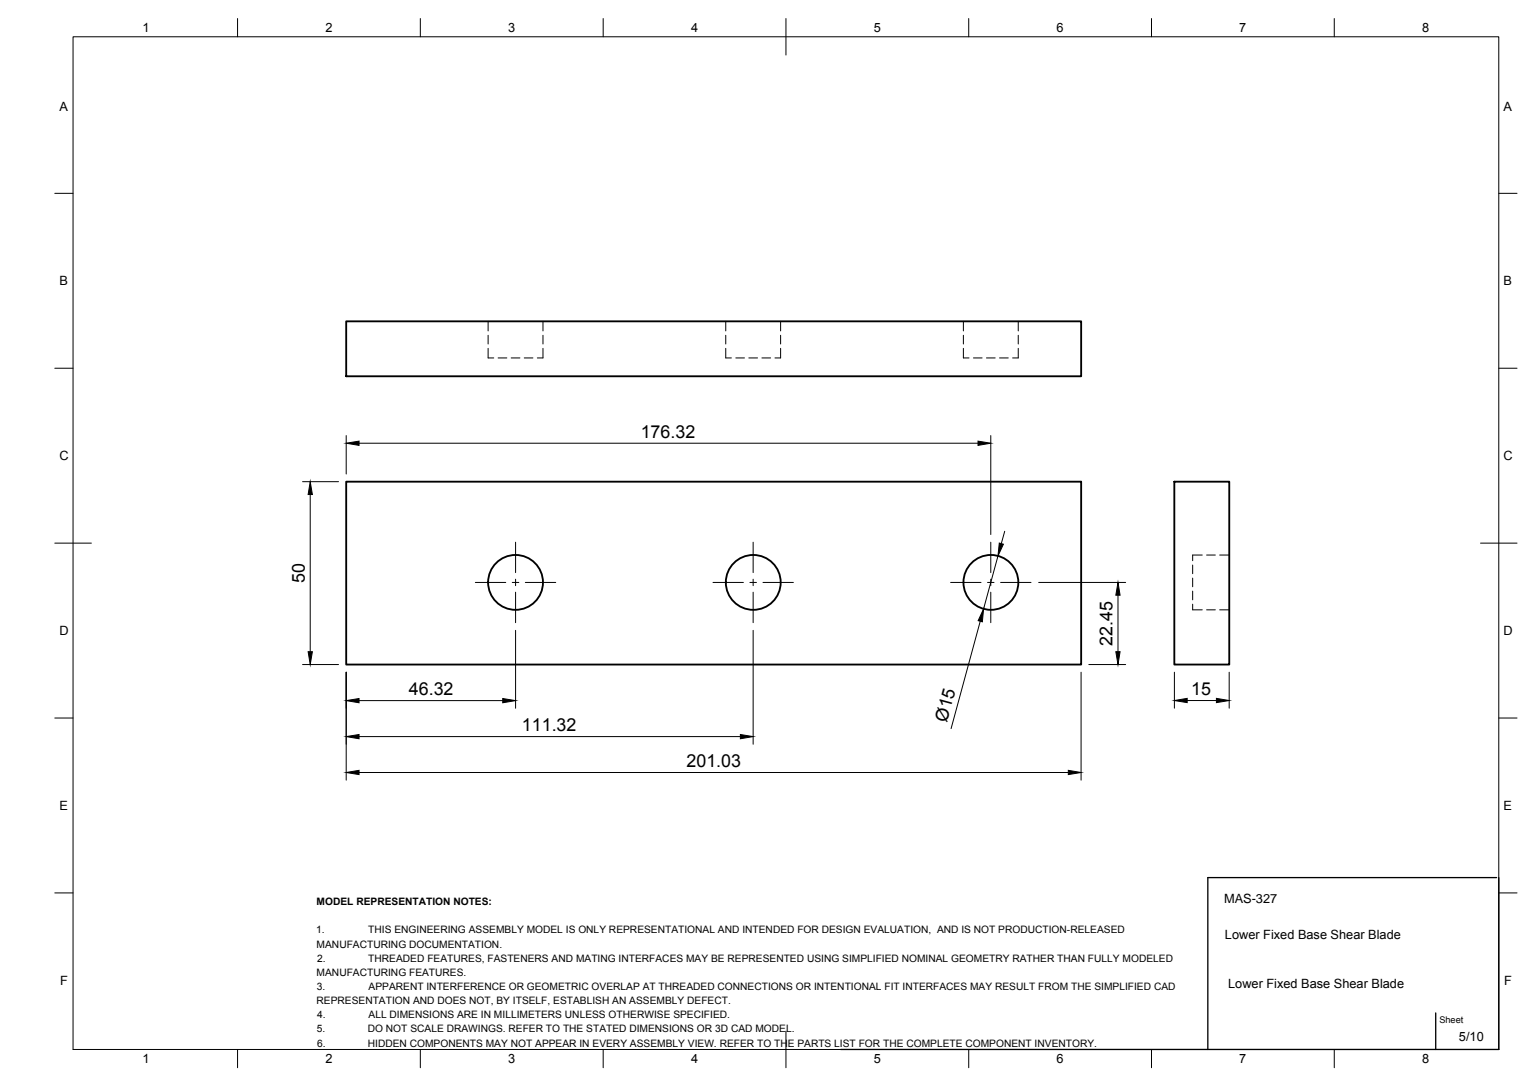
ISO-10303-21;
HEADER;
FILE_DESCRIPTION (('STEP AP214'),
    '1' );
FILE_NAME ('Lower Fixed Base Shear Blade.step',
    '2026-10-06T22:16:42',
    ( '' ),
    ( '' ),
    'SwSTEP 2.0',
    'SolidWorks 2025',
    '' );
FILE_SCHEMA (( 'AUTOMOTIVE_DESIGN' ));
ENDSEC;

DATA;
#67=AXIS2_PLACEMENT_3D ( 'NONE', #12131, #8413, #1572 ) ;
#82=DIRECTION ( 'NONE',  ( 0.000000000000000000, 0.000000000000000000, -1.000000000000000000 ) ) ;
#121=EDGE_CURVE ( 'NONE', #811, #5132, #2980, .T. ) ;
#220=CARTESIAN_POINT ( 'NONE',  ( 83.67254549292280785, -61.68114226949890622, 10.00000000000001599 ) ) ;
#222=ORIENTED_EDGE ( 'NONE', *, *, #8399, .T. ) ;
#275=CARTESIAN_POINT ( 'NONE',  ( 173.3794444120442506, -34.13255853780189142, 5.000000000000018652 ) ) ;
#342=EDGE_CURVE ( 'NONE', #19257, #8316, #5649, .T. ) ;
#343=( GEOMETRIC_REPRESENTATION_CONTEXT ( 3 ) GLOBAL_UNCERTAINTY_ASSIGNED_CONTEXT ( ( #15680 ) ) GLOBAL_UNIT_ASSIGNED_CONTEXT ( ( #12211, #2186, #7269 ) ) REPRESENTATION_CONTEXT ( 'NONE', 'WORKASPACE' ) );
#363=CARTESIAN_POINT ( 'NONE',  ( 18.67254549292281496, -61.68114226949890622, 10.00000000000001599 ) ) ;
#364=EDGE_CURVE ( 'NONE', #13608, #15461, #11277, .T. ) ;
#394=LINE ( 'NONE', #7017, #18876 ) ;
#660=EDGE_CURVE ( 'NONE', #15106, #2386, #14957, .T. ) ;
#672=LINE ( 'NONE', #7408, #19081 ) ;
#751=DIRECTION ( 'NONE',  ( 1.000000000000000000, 0.000000000000000000, 0.000000000000000000 ) ) ;
#771=AXIS2_PLACEMENT_3D ( 'NONE', #11380, #1580, #9853 ) ;
#811=VERTEX_POINT ( 'NONE', #13743 ) ;
#889=DIRECTION ( 'NONE',  ( 1.000000000000000000, -0.000000000000000000, -0.000000000000000000 ) ) ;
#892=EDGE_LOOP ( 'NONE', ( #21201, #9511, #8668, #6236 ) ) ;
#909=CARTESIAN_POINT ( 'NONE',  ( -27.64582385433944367, -84.13255853780189852, 5.000000000000018652 ) ) ;
#912=EDGE_LOOP ( 'NONE', ( #15164, #18877, #13960, #16804 ) ) ;
#919=CARTESIAN_POINT ( 'NONE',  ( 5.130598475945862827E-15, 0.000000000000000000, 20.00000000000001776 ) ) ;
#928=AXIS2_PLACEMENT_3D ( 'NONE', #10600, #15343, #18757 ) ;
#1190=PLANE ( 'NONE',  #6786 ) ;
#1247=FACE_OUTER_BOUND ( 'NONE', #20004, .T. ) ;
#1249=VERTEX_POINT ( 'NONE', #14943 ) ;
#1316=CARTESIAN_POINT ( 'NONE',  ( 18.67254549292281496, -61.68114226949890622, -16.21320343559643717 ) ) ;
#1428=CYLINDRICAL_SURFACE ( 'NONE', #9034, 7.500000000000000000 ) ;
#1449=ORIENTED_EDGE ( 'NONE', *, *, #19445, .T. ) ;
#1456=CARTESIAN_POINT ( 'NONE',  ( 83.67254549292280785, -61.68114226949890622, -16.21320343559643717 ) ) ;
#1481=CIRCLE ( 'NONE', #2895, 7.500000000000000000 ) ;
#1565=CIRCLE ( 'NONE', #17047, 7.500000000000007105 ) ;
#1572=DIRECTION ( 'NONE',  ( -1.000000000000000000, 0.000000000000000000, 0.000000000000000000 ) ) ;
#1580=DIRECTION ( 'NONE',  ( -0.000000000000000000, 0.000000000000000000, -1.000000000000000000 ) ) ;
#1638=DIRECTION ( 'NONE',  ( -0.000000000000000000, -0.000000000000000000, 1.000000000000000000 ) ) ;
#1724=FACE_OUTER_BOUND ( 'NONE', #3351, .T. ) ;
#1788=CARTESIAN_POINT ( 'NONE',  ( -27.64582385433943656, -34.13255853780189142, 5.000000000000018652 ) ) ;
#1876=DIRECTION ( 'NONE',  ( -0.000000000000000000, -0.000000000000000000, -1.000000000000000000 ) ) ;
#1912=CARTESIAN_POINT ( 'NONE',  ( 173.3794444120442506, -34.13255853780189142, 5.000000000000018652 ) ) ;
#2073=ORIENTED_EDGE ( 'NONE', *, *, #13532, .T. ) ;
#2131=CLOSED_SHELL ( 'NONE', ( #14070, #2497, #19372, #16215, #5248, #3409, #5840, #17907, #3304, #2907, #15780, #10582, #17008, #14366, #6702 ) ) ;
#2151=FILL_AREA_STYLE_COLOUR ( '', #21717 ) ;
#2186=( NAMED_UNIT ( * ) PLANE_ANGLE_UNIT ( ) SI_UNIT ( $, .RADIAN. ) );
#2350=STYLED_ITEM ( 'NONE', ( #2362 ), #14370 ) ;
#2362=PRESENTATION_STYLE_ASSIGNMENT (( #17561 ) ) ;
#2386=VERTEX_POINT ( 'NONE', #5094 ) ;
#2403=CARTESIAN_POINT ( 'NONE',  ( 0.000000000000000000, 0.000000000000000000, 0.000000000000000000 ) ) ;
#2410=DIRECTION ( 'NONE',  ( 1.387778780781445676E-16, 1.000000000000000000, -0.000000000000000000 ) ) ;
#2433=CARTESIAN_POINT ( 'NONE',  ( 173.3794444120442506, -34.13255853780189142, 5.000000000000018652 ) ) ;
#2489=AXIS2_PLACEMENT_3D ( 'NONE', #220, #19066, #12443 ) ;
#2497=ADVANCED_FACE ( 'NONE', ( #6651 ), #18088, .F. ) ;
#2515=DIRECTION ( 'NONE',  ( -1.000000000000000000, 0.000000000000000000, 0.000000000000000000 ) ) ;
#2644=ORIENTED_EDGE ( 'NONE', *, *, #20541, .F. ) ;
#2725=DIRECTION ( 'NONE',  ( -0.000000000000000000, -0.000000000000000000, -1.000000000000000000 ) ) ;
#2788=ORIENTED_EDGE ( 'NONE', *, *, #16877, .F. ) ;
#2846=DIRECTION ( 'NONE',  ( -0.000000000000000000, -0.000000000000000000, 1.000000000000000000 ) ) ;
#2895=AXIS2_PLACEMENT_3D ( 'NONE', #5494, #19276, #2515 ) ;
#2907=ADVANCED_FACE ( 'NONE', ( #16405 ), #1428, .F. ) ;
#2908=( NAMED_UNIT ( * ) PLANE_ANGLE_UNIT ( ) SI_UNIT ( $, .RADIAN. ) );
#2926=CARTESIAN_POINT ( 'NONE',  ( 156.1725454929228079, -61.68114226949890622, -16.21320343559643717 ) ) ;
#2949=DIRECTION ( 'NONE',  ( -1.000000000000000000, 0.000000000000000000, 0.000000000000000000 ) ) ;
#2980=LINE ( 'NONE', #6398, #9178 ) ;
#3181=ORIENTED_EDGE ( 'NONE', *, *, #12830, .F. ) ;
#3202=ORIENTED_EDGE ( 'NONE', *, *, #14985, .T. ) ;
#3219=DIRECTION ( 'NONE',  ( 1.000000000000000000, 0.000000000000000000, 0.000000000000000000 ) ) ;
#3304=ADVANCED_FACE ( 'NONE', ( #16007, #13043, #19880, #9417 ), #4433, .F. ) ;
#3351=EDGE_LOOP ( 'NONE', ( #5084, #7985, #17552, #7309 ) ) ;
#3409=ADVANCED_FACE ( 'NONE', ( #11003 ), #15954, .F. ) ;
#3434=DIRECTION ( 'NONE',  ( -1.000000000000000000, 0.000000000000000000, 0.000000000000000000 ) ) ;
#3438=ORIENTED_EDGE ( 'NONE', *, *, #5810, .F. ) ;
#3566=EDGE_CURVE ( 'NONE', #5132, #8905, #20825, .T. ) ;
#3874=CARTESIAN_POINT ( 'NONE',  ( 156.1725454929228079, -61.68114226949890622, 20.00000000000001776 ) ) ;
#3887=DIRECTION ( 'NONE',  ( 0.000000000000000000, 0.000000000000000000, 1.000000000000000000 ) ) ;
#4020=EDGE_LOOP ( 'NONE', ( #19518, #2644, #17019, #15348 ) ) ;
#4101=VECTOR ( 'NONE', #5859, 1000.000000000000000 ) ;
#4120=EDGE_LOOP ( 'NONE', ( #9807, #20346, #10050, #6259 ) ) ;
#4123=CARTESIAN_POINT ( 'NONE',  ( 173.3794444120442506, -34.13255853780189142, 5.000000000000018652 ) ) ;
#4141=SHAPE_DEFINITION_REPRESENTATION ( #21024, #13805 ) ;
#4194=CARTESIAN_POINT ( 'NONE',  ( 83.67254549292280785, -61.68114226949890622, 20.00000000000001776 ) ) ;
#4321=DIRECTION ( 'NONE',  ( 0.000000000000000000, -0.000000000000000000, 1.000000000000000000 ) ) ;
#4328=EDGE_LOOP ( 'NONE', ( #1449, #19360 ) ) ;
#4433=PLANE ( 'NONE',  #4787 ) ;
#4635=ORIENTED_EDGE ( 'NONE', *, *, #3566, .T. ) ;
#4643=AXIS2_PLACEMENT_3D ( 'NONE', #13010, #19731, #5950 ) ;
#4664=DIRECTION ( 'NONE',  ( -1.000000000000000000, 0.000000000000000000, 0.000000000000000000 ) ) ;
#4787=AXIS2_PLACEMENT_3D ( 'NONE', #919, #12819, #4664 ) ;
#4828=LINE ( 'NONE', #8146, #19281 ) ;
#4912=DIRECTION ( 'NONE',  ( -0.000000000000000000, -0.000000000000000000, 1.000000000000000000 ) ) ;
#5084=ORIENTED_EDGE ( 'NONE', *, *, #660, .F. ) ;
#5094=CARTESIAN_POINT ( 'NONE',  ( 156.1725454929228079, -61.68114226949890622, 10.00000000000001599 ) ) ;
#5132=VERTEX_POINT ( 'NONE', #909 ) ;
#5248=ADVANCED_FACE ( 'NONE', ( #5976 ), #19424, .F. ) ;
#5397=ORIENTED_EDGE ( 'NONE', *, *, #6235, .T. ) ;
#5413=PLANE ( 'NONE',  #67 ) ;
#5494=CARTESIAN_POINT ( 'NONE',  ( 18.67254549292281496, -61.68114226949890622, 20.00000000000001776 ) ) ;
#5516=VERTEX_POINT ( 'NONE', #10279 ) ;
#5552=ORIENTED_EDGE ( 'NONE', *, *, #342, .F. ) ;
#5643=EDGE_CURVE ( 'NONE', #15461, #6487, #672, .T. ) ;
#5649=CIRCLE ( 'NONE', #17965, 7.500000000000000000 ) ;
#5656=ORIENTED_EDGE ( 'NONE', *, *, #11935, .T. ) ;
#5664=LINE ( 'NONE', #13929, #16586 ) ;
#5708=DIRECTION ( 'NONE',  ( -0.000000000000000000, -0.000000000000000000, 1.000000000000000000 ) ) ;
#5784=PRODUCT_CONTEXT ( 'NONE', #7051, 'mechanical' ) ;
#5810=EDGE_CURVE ( 'NONE', #1249, #19734, #14847, .T. ) ;
#5840=ADVANCED_FACE ( 'NONE', ( #20366 ), #18813, .F. ) ;
#5859=DIRECTION ( 'NONE',  ( 1.000000000000000000, -0.000000000000000000, -0.000000000000000000 ) ) ;
#5950=DIRECTION ( 'NONE',  ( -1.000000000000000000, 0.000000000000000000, 0.000000000000000000 ) ) ;
#5976=FACE_OUTER_BOUND ( 'NONE', #4020, .T. ) ;
#5989=FACE_OUTER_BOUND ( 'NONE', #10586, .T. ) ;
#5995=CARTESIAN_POINT ( 'NONE',  ( 11.17254549292281673, -61.68114226949890622, -16.21320343559643717 ) ) ;
#6192=DIRECTION ( 'NONE',  ( 0.000000000000000000, 1.000000000000000000, 0.000000000000000000 ) ) ;
#6235=EDGE_CURVE ( 'NONE', #8905, #7289, #13727, .T. ) ;
#6236=ORIENTED_EDGE ( 'NONE', *, *, #14985, .F. ) ;
#6259=ORIENTED_EDGE ( 'NONE', *, *, #16877, .T. ) ;
#6260=DIRECTION ( 'NONE',  ( -0.000000000000000000, -0.000000000000000000, 1.000000000000000000 ) ) ;
#6272=DIRECTION ( 'NONE',  ( -0.000000000000000000, -0.000000000000000000, 1.000000000000000000 ) ) ;
#6331=DIRECTION ( 'NONE',  ( -1.000000000000000000, 0.000000000000000000, 0.000000000000000000 ) ) ;
#6398=CARTESIAN_POINT ( 'NONE',  ( 173.3794444120442506, -84.13255853780189852, 5.000000000000018652 ) ) ;
#6487=VERTEX_POINT ( 'NONE', #10965 ) ;
#6494=LINE ( 'NONE', #21381, #19691 ) ;
#6553=CARTESIAN_POINT ( 'NONE',  ( 83.67254549292280785, -61.68114226949890622, -16.21320343559643717 ) ) ;
#6579=AXIS2_PLACEMENT_3D ( 'NONE', #4194, #16191, #21066 ) ;
#6582=MECHANICAL_DESIGN_GEOMETRIC_PRESENTATION_REPRESENTATION('',(#2350),#18555);
#6651=FACE_OUTER_BOUND ( 'NONE', #8147, .T. ) ;
#6696=DIRECTION ( 'NONE',  ( 1.000000000000000000, 0.000000000000000000, 0.000000000000000000 ) ) ;
#6702=ADVANCED_FACE ( 'NONE', ( #7778 ), #17889, .F. ) ;
#6771=VECTOR ( 'NONE', #18889, 1000.000000000000000 ) ;
#6780=EDGE_LOOP ( 'NONE', ( #20219, #9123 ) ) ;
#6786=AXIS2_PLACEMENT_3D ( 'NONE', #7602, #21047, #2949 ) ;
#6907=CARTESIAN_POINT ( 'NONE',  ( 173.3794444120442506, -84.13255853780189852, 5.000000000000018652 ) ) ;
#6932=VERTEX_POINT ( 'NONE', #1912 ) ;
#6959=EDGE_LOOP ( 'NONE', ( #2073, #2788, #11632, #5397 ) ) ;
#6962=ORIENTED_EDGE ( 'NONE', *, *, #15169, .F. ) ;
#7017=CARTESIAN_POINT ( 'NONE',  ( -27.64582385433943656, -34.13255853780189142, 20.00000000000001776 ) ) ;
#7050=DIRECTION ( 'NONE',  ( 0.000000000000000000, 0.000000000000000000, 1.000000000000000000 ) ) ;
#7051=APPLICATION_CONTEXT ( 'automotive_design' ) ;
#7122=DIRECTION ( 'NONE',  ( -0.000000000000000000, -0.000000000000000000, 1.000000000000000000 ) ) ;
#7130=CARTESIAN_POINT ( 'NONE',  ( -27.64582385433943656, -34.13255853780189142, 5.000000000000018652 ) ) ;
#7233=SURFACE_STYLE_FILL_AREA ( #17235 ) ;
#7269=( NAMED_UNIT ( * ) SI_UNIT ( $, .STERADIAN. ) SOLID_ANGLE_UNIT ( ) );
#7289=VERTEX_POINT ( 'NONE', #18172 ) ;
#7309=ORIENTED_EDGE ( 'NONE', *, *, #8399, .F. ) ;
#7408=CARTESIAN_POINT ( 'NONE',  ( 76.17254549292280785, -61.68114226949890622, -16.21320343559643717 ) ) ;
#7602=CARTESIAN_POINT ( 'NONE',  ( 5.130598475945862827E-15, 0.000000000000000000, 5.000000000000018652 ) ) ;
#7608=CARTESIAN_POINT ( 'NONE',  ( 141.1725454929228079, -61.68114226949890622, 10.00000000000001599 ) ) ;
#7712=DIRECTION ( 'NONE',  ( 1.387778780781445676E-16, 1.000000000000000000, 0.000000000000000000 ) ) ;
#7778=FACE_OUTER_BOUND ( 'NONE', #9885, .T. ) ;
#7833=CARTESIAN_POINT ( 'NONE',  ( 83.67254549292280785, -61.68114226949890622, 10.00000000000001599 ) ) ;
#7938=DIRECTION ( 'NONE',  ( -1.000000000000000000, 0.000000000000000000, 0.000000000000000000 ) ) ;
#7985=ORIENTED_EDGE ( 'NONE', *, *, #12830, .T. ) ;
#8013=PRODUCT ( 'Lower Fixed Base Shear Blade', 'Lower Fixed Base Shear Blade', '', ( #5784 ) ) ;
#8146=CARTESIAN_POINT ( 'NONE',  ( 141.1725454929228079, -61.68114226949890622, -16.21320343559643717 ) ) ;
#8147=EDGE_LOOP ( 'NONE', ( #17763, #14172, #16091, #14849 ) ) ;
#8307=APPLICATION_CONTEXT ( 'automotive_design' ) ;
#8316=VERTEX_POINT ( 'NONE', #13175 ) ;
#8365=ORIENTED_EDGE ( 'NONE', *, *, #14042, .F. ) ;
#8399=EDGE_CURVE ( 'NONE', #2386, #18846, #11293, .T. ) ;
#8413=DIRECTION ( 'NONE',  ( -0.000000000000000000, 0.000000000000000000, -1.000000000000000000 ) ) ;
#8485=LINE ( 'NONE', #18612, #11937 ) ;
#8532=AXIS2_PLACEMENT_3D ( 'NONE', #13473, #8629, #15238 ) ;
#8629=DIRECTION ( 'NONE',  ( 0.000000000000000000, 0.000000000000000000, 1.000000000000000000 ) ) ;
#8641=ORIENTED_EDGE ( 'NONE', *, *, #15855, .T. ) ;
#8668=ORIENTED_EDGE ( 'NONE', *, *, #17575, .F. ) ;
#8688=VECTOR ( 'NONE', #2410, 1000.000000000000000 ) ;
#8728=AXIS2_PLACEMENT_3D ( 'NONE', #16220, #6192, #4321 ) ;
#8749=ORIENTED_EDGE ( 'NONE', *, *, #15855, .F. ) ;
#8777=DIRECTION ( 'NONE',  ( -0.000000000000000000, -0.000000000000000000, 1.000000000000000000 ) ) ;
#8884=SURFACE_SIDE_STYLE ('',( #7233 ) ) ;
#8891=AXIS2_PLACEMENT_3D ( 'NONE', #21113, #19550, #18112 ) ;
#8905=VERTEX_POINT ( 'NONE', #1788 ) ;
#9034=AXIS2_PLACEMENT_3D ( 'NONE', #1316, #6272, #18059 ) ;
#9095=ORIENTED_EDGE ( 'NONE', *, *, #15940, .T. ) ;
#9116=EDGE_CURVE ( 'NONE', #17048, #18846, #17863, .T. ) ;
#9123=ORIENTED_EDGE ( 'NONE', *, *, #17267, .T. ) ;
#9178=VECTOR ( 'NONE', #17963, 1000.000000000000000 ) ;
#9185=CARTESIAN_POINT ( 'NONE',  ( 91.17254549292282206, -61.68114226949890622, 10.00000000000001599 ) ) ;
#9230=ORIENTED_EDGE ( 'NONE', *, *, #342, .T. ) ;
#9259=EDGE_CURVE ( 'NONE', #6487, #12008, #20656, .T. ) ;
#9379=VECTOR ( 'NONE', #7122, 1000.000000000000000 ) ;
#9417=FACE_OUTER_BOUND ( 'NONE', #13271, .T. ) ;
#9425=AXIS2_PLACEMENT_3D ( 'NONE', #13165, #14917, #6331 ) ;
#9511=ORIENTED_EDGE ( 'NONE', *, *, #21604, .T. ) ;
#9680=SHAPE_REPRESENTATION_RELATIONSHIP ( 'NONE' , 'NONE' ,  #13805, #13742 ) ;
#9701=DIRECTION ( 'NONE',  ( 0.000000000000000000, -1.000000000000000000, 0.000000000000000000 ) ) ;
#9749=CARTESIAN_POINT ( 'NONE',  ( 141.1725454929228079, -61.68114226949890622, 20.00000000000001776 ) ) ;
#9803=DIRECTION ( 'NONE',  ( 0.000000000000000000, 0.000000000000000000, 1.000000000000000000 ) ) ;
#9807=ORIENTED_EDGE ( 'NONE', *, *, #15169, .T. ) ;
#9853=DIRECTION ( 'NONE',  ( -1.000000000000000000, 0.000000000000000000, 0.000000000000000000 ) ) ;
#9858=ORIENTED_EDGE ( 'NONE', *, *, #121, .T. ) ;
#9885=EDGE_LOOP ( 'NONE', ( #8641, #14747 ) ) ;
#9912=LINE ( 'NONE', #16503, #18987 ) ;
#9923=CIRCLE ( 'NONE', #20482, 7.500000000000000000 ) ;
#10047=CARTESIAN_POINT ( 'NONE',  ( 18.67254549292281496, -61.68114226949890622, 20.00000000000001776 ) ) ;
#10050=ORIENTED_EDGE ( 'NONE', *, *, #21369, .F. ) ;
#10119=CIRCLE ( 'NONE', #18564, 7.500000000000007105 ) ;
#10279=CARTESIAN_POINT ( 'NONE',  ( 173.3794444120442506, -34.13255853780189142, 20.00000000000001776 ) ) ;
#10399=CARTESIAN_POINT ( 'NONE',  ( -27.64582385433944367, -84.13255853780189852, 20.00000000000001776 ) ) ;
#10428=LINE ( 'NONE', #6907, #9379 ) ;
#10582=ADVANCED_FACE ( 'NONE', ( #17888 ), #14806, .F. ) ;
#10586=EDGE_LOOP ( 'NONE', ( #3181, #8749, #222, #18771 ) ) ;
#10600=CARTESIAN_POINT ( 'NONE',  ( 148.6725454929228079, -61.68114226949890622, 20.00000000000001776 ) ) ;
#10613=ORIENTED_EDGE ( 'NONE', *, *, #364, .T. ) ;
#10647=VECTOR ( 'NONE', #6260, 1000.000000000000000 ) ;
#10795=CARTESIAN_POINT ( 'NONE',  ( -27.64582385433943656, -34.13255853780189142, 5.000000000000018652 ) ) ;
#10858=DIRECTION ( 'NONE',  ( -0.000000000000000000, -0.000000000000000000, 1.000000000000000000 ) ) ;
#10965=CARTESIAN_POINT ( 'NONE',  ( 76.17254549292280785, -61.68114226949890622, 20.00000000000001776 ) ) ;
#10988=AXIS2_PLACEMENT_3D ( 'NONE', #12188, #20688, #82 ) ;
#11003=FACE_OUTER_BOUND ( 'NONE', #11770, .T. ) ;
#11055=AXIS2_PLACEMENT_3D ( 'NONE', #14405, #5708, #751 ) ;
#11067=DIRECTION ( 'NONE',  ( -0.000000000000000000, -0.000000000000000000, 1.000000000000000000 ) ) ;
#11114=EDGE_CURVE ( 'NONE', #15461, #13608, #10119, .T. ) ;
#11277=CIRCLE ( 'NONE', #2489, 7.500000000000007105 ) ;
#11293=LINE ( 'NONE', #2926, #15056 ) ;
#11380=CARTESIAN_POINT ( 'NONE',  ( 5.130598475945862827E-15, 0.000000000000000000, 10.00000000000001599 ) ) ;
#11608=ORIENTED_EDGE ( 'NONE', *, *, #17575, .T. ) ;
#11610=ORIENTED_EDGE ( 'NONE', *, *, #13532, .F. ) ;
#11632=ORIENTED_EDGE ( 'NONE', *, *, #15940, .F. ) ;
#11770=EDGE_LOOP ( 'NONE', ( #15079, #21540, #14501, #21735 ) ) ;
#11808=AXIS2_PLACEMENT_3D ( 'NONE', #18274, #9803, #19597 ) ;
#11935=EDGE_CURVE ( 'NONE', #12008, #6487, #15418, .T. ) ;
#11937=VECTOR ( 'NONE', #1638, 1000.000000000000000 ) ;
#12008=VERTEX_POINT ( 'NONE', #21552 ) ;
#12131=CARTESIAN_POINT ( 'NONE',  ( 5.130598475945862827E-15, 0.000000000000000000, 10.00000000000001599 ) ) ;
#12188=CARTESIAN_POINT ( 'NONE',  ( 173.3794444120442506, -34.13255853780189142, 5.000000000000018652 ) ) ;
#12211=( LENGTH_UNIT ( ) NAMED_UNIT ( * ) SI_UNIT ( .MILLI., .METRE. ) );
#12252=DIRECTION ( 'NONE',  ( -1.000000000000000000, 0.000000000000000000, 0.000000000000000000 ) ) ;
#12392=DIRECTION ( 'NONE',  ( -0.000000000000000000, -0.000000000000000000, 1.000000000000000000 ) ) ;
#12443=DIRECTION ( 'NONE',  ( -1.000000000000000000, 0.000000000000000000, 0.000000000000000000 ) ) ;
#12470=ORIENTED_EDGE ( 'NONE', *, *, #11114, .T. ) ;
#12657=AXIS2_PLACEMENT_3D ( 'NONE', #2403, #7050, #17169 ) ;
#12770=CARTESIAN_POINT ( 'NONE',  ( 26.17254549292281496, -61.68114226949890622, -16.21320343559643717 ) ) ;
#12819=DIRECTION ( 'NONE',  ( -0.000000000000000000, 0.000000000000000000, -1.000000000000000000 ) ) ;
#12830=EDGE_CURVE ( 'NONE', #15106, #17048, #4828, .T. ) ;
#13010=CARTESIAN_POINT ( 'NONE',  ( 18.67254549292281496, -61.68114226949890622, 10.00000000000001599 ) ) ;
#13043=FACE_BOUND ( 'NONE', #18393, .T. ) ;
#13165=CARTESIAN_POINT ( 'NONE',  ( 83.67254549292280785, -61.68114226949890622, 20.00000000000001776 ) ) ;
#13175=CARTESIAN_POINT ( 'NONE',  ( 26.17254549292281496, -61.68114226949890622, 20.00000000000001776 ) ) ;
#13192=CARTESIAN_POINT ( 'NONE',  ( 11.17254549292281673, -61.68114226949890622, 10.00000000000001599 ) ) ;
#13198=DIRECTION ( 'NONE',  ( -0.000000000000000000, 0.000000000000000000, 1.000000000000000000 ) ) ;
#13269=VERTEX_POINT ( 'NONE', #15252 ) ;
#13271=EDGE_LOOP ( 'NONE', ( #6962, #11610, #8365, #14546 ) ) ;
#13473=CARTESIAN_POINT ( 'NONE',  ( 148.6725454929228079, -61.68114226949890622, 10.00000000000001599 ) ) ;
#13512=CARTESIAN_POINT ( 'NONE',  ( 148.6725454929228079, -61.68114226949890622, -16.21320343559643717 ) ) ;
#13532=EDGE_CURVE ( 'NONE', #7289, #5516, #17535, .T. ) ;
#13608=VERTEX_POINT ( 'NONE', #9185 ) ;
#13727=LINE ( 'NONE', #7130, #15550 ) ;
#13742=ADVANCED_BREP_SHAPE_REPRESENTATION ( '', ( #14370, #12657 ), #343 ) ;
#13743=CARTESIAN_POINT ( 'NONE',  ( 173.3794444120442506, -84.13255853780189852, 5.000000000000018652 ) ) ;
#13805=SHAPE_REPRESENTATION ( 'Lower Fixed Base Shear Blade', ( #12657 ), #343 ) ;
#13829=CYLINDRICAL_SURFACE ( 'NONE', #15706, 7.500000000000007105 ) ;
#13929=CARTESIAN_POINT ( 'NONE',  ( 173.3794444120442506, -84.13255853780189852, 20.00000000000001776 ) ) ;
#13960=ORIENTED_EDGE ( 'NONE', *, *, #20210, .T. ) ;
#14042=EDGE_CURVE ( 'NONE', #17319, #7289, #394, .T. ) ;
#14052=EDGE_CURVE ( 'NONE', #811, #13269, #10428, .T. ) ;
#14070=ADVANCED_FACE ( 'NONE', ( #1724 ), #13829, .F. ) ;
#14088=CARTESIAN_POINT ( 'NONE',  ( -27.64582385433943656, -34.13255853780189142, 5.000000000000018652 ) ) ;
#14172=ORIENTED_EDGE ( 'NONE', *, *, #5643, .T. ) ;
#14188=CARTESIAN_POINT ( 'NONE',  ( 148.6725454929228079, -61.68114226949890622, 20.00000000000001776 ) ) ;
#14330=LINE ( 'NONE', #2433, #18726 ) ;
#14366=ADVANCED_FACE ( 'NONE', ( #5989 ), #17453, .F. ) ;
#14370=MANIFOLD_SOLID_BREP ( 'Body-Move/Copy1', #2131 ) ;
#14405=CARTESIAN_POINT ( 'NONE',  ( 18.67254549292281496, -61.68114226949890622, -16.21320343559643717 ) ) ;
#14501=ORIENTED_EDGE ( 'NONE', *, *, #3566, .F. ) ;
#14546=ORIENTED_EDGE ( 'NONE', *, *, #16615, .F. ) ;
#14666=AXIS2_PLACEMENT_3D ( 'NONE', #19229, #12392, #19127 ) ;
#14747=ORIENTED_EDGE ( 'NONE', *, *, #660, .T. ) ;
#14806=CYLINDRICAL_SURFACE ( 'NONE', #21377, 7.500000000000007105 ) ;
#14847=CIRCLE ( 'NONE', #4643, 7.500000000000000000 ) ;
#14849=ORIENTED_EDGE ( 'NONE', *, *, #20210, .F. ) ;
#14890=DIRECTION ( 'NONE',  ( -0.000000000000000000, -0.000000000000000000, 1.000000000000000000 ) ) ;
#14917=DIRECTION ( 'NONE',  ( -0.000000000000000000, -0.000000000000000000, -1.000000000000000000 ) ) ;
#14943=CARTESIAN_POINT ( 'NONE',  ( 26.17254549292281496, -61.68114226949890622, 10.00000000000001599 ) ) ;
#14957=CIRCLE ( 'NONE', #11808, 7.500000000000007105 ) ;
#14985=EDGE_CURVE ( 'NONE', #1249, #8316, #16392, .T. ) ;
#14995=AXIS2_PLACEMENT_3D ( 'NONE', #14088, #17822, #7712 ) ;
#15056=VECTOR ( 'NONE', #4912, 1000.000000000000000 ) ;
#15079=ORIENTED_EDGE ( 'NONE', *, *, #14042, .T. ) ;
#15106=VERTEX_POINT ( 'NONE', #7608 ) ;
#15164=ORIENTED_EDGE ( 'NONE', *, *, #5643, .F. ) ;
#15169=EDGE_CURVE ( 'NONE', #5516, #13269, #18462, .T. ) ;
#15236=PRODUCT_DEFINITION_CONTEXT ( 'detailed design', #8307, 'design' ) ;
#15238=DIRECTION ( 'NONE',  ( -1.000000000000000000, 0.000000000000000000, 0.000000000000000000 ) ) ;
#15252=CARTESIAN_POINT ( 'NONE',  ( 173.3794444120442506, -84.13255853780189852, 20.00000000000001776 ) ) ;
#15343=DIRECTION ( 'NONE',  ( -0.000000000000000000, -0.000000000000000000, -1.000000000000000000 ) ) ;
#15348=ORIENTED_EDGE ( 'NONE', *, *, #14052, .T. ) ;
#15418=CIRCLE ( 'NONE', #9425, 7.500000000000007105 ) ;
#15461=VERTEX_POINT ( 'NONE', #19760 ) ;
#15550=VECTOR ( 'NONE', #20463, 1000.000000000000000 ) ;
#15583=FACE_OUTER_BOUND ( 'NONE', #4120, .T. ) ;
#15680=UNCERTAINTY_MEASURE_WITH_UNIT (LENGTH_MEASURE( 1.000000000000000082E-05 ), #12211, 'distance_accuracy_value', 'NONE');
#15706=AXIS2_PLACEMENT_3D ( 'NONE', #13512, #8777, #6696 ) ;
#15780=ADVANCED_FACE ( 'NONE', ( #20526 ), #5413, .F. ) ;
#15840=CYLINDRICAL_SURFACE ( 'NONE', #11055, 7.500000000000000000 ) ;
#15855=EDGE_CURVE ( 'NONE', #2386, #15106, #17293, .T. ) ;
#15893=VECTOR ( 'NONE', #10858, 1000.000000000000000 ) ;
#15940=EDGE_CURVE ( 'NONE', #8905, #6932, #14330, .T. ) ;
#15954=PLANE ( 'NONE',  #14995 ) ;
#16007=FACE_BOUND ( 'NONE', #4328, .T. ) ;
#16091=ORIENTED_EDGE ( 'NONE', *, *, #11935, .F. ) ;
#16191=DIRECTION ( 'NONE',  ( -0.000000000000000000, -0.000000000000000000, -1.000000000000000000 ) ) ;
#16215=ADVANCED_FACE ( 'NONE', ( #15583 ), #18685, .F. ) ;
#16220=CARTESIAN_POINT ( 'NONE',  ( 173.3794444120442506, -84.13255853780189852, 5.000000000000018652 ) ) ;
#16297=DIRECTION ( 'NONE',  ( 0.000000000000000000, 0.000000000000000000, 1.000000000000000000 ) ) ;
#16392=LINE ( 'NONE', #12770, #10647 ) ;
#16405=FACE_OUTER_BOUND ( 'NONE', #18586, .T. ) ;
#16457=LINE ( 'NONE', #5995, #17567 ) ;
#16503=CARTESIAN_POINT ( 'NONE',  ( 91.17254549292282206, -61.68114226949890622, -16.21320343559643717 ) ) ;
#16563=DIRECTION ( 'NONE',  ( -0.000000000000000000, -0.000000000000000000, 1.000000000000000000 ) ) ;
#16586=VECTOR ( 'NONE', #20564, 1000.000000000000000 ) ;
#16615=EDGE_CURVE ( 'NONE', #13269, #17319, #5664, .T. ) ;
#16804=ORIENTED_EDGE ( 'NONE', *, *, #9259, .F. ) ;
#16877=EDGE_CURVE ( 'NONE', #6932, #5516, #21104, .T. ) ;
#17008=ADVANCED_FACE ( 'NONE', ( #1247 ), #19768, .F. ) ;
#17019=ORIENTED_EDGE ( 'NONE', *, *, #121, .F. ) ;
#17047=AXIS2_PLACEMENT_3D ( 'NONE', #14188, #2725, #20927 ) ;
#17048=VERTEX_POINT ( 'NONE', #9749 ) ;
#17119=CARTESIAN_POINT ( 'NONE',  ( 173.3794444120442506, -34.13255853780189142, 20.00000000000001776 ) ) ;
#17169=DIRECTION ( 'NONE',  ( 1.000000000000000000, 0.000000000000000000, 0.000000000000000000 ) ) ;
#17235=FILL_AREA_STYLE ('',( #2151 ) ) ;
#17267=EDGE_CURVE ( 'NONE', #19734, #1249, #9923, .T. ) ;
#17293=CIRCLE ( 'NONE', #8532, 7.500000000000007105 ) ;
#17319=VERTEX_POINT ( 'NONE', #10399 ) ;
#17346=ORIENTED_EDGE ( 'NONE', *, *, #9259, .T. ) ;
#17453=CYLINDRICAL_SURFACE ( 'NONE', #14666, 7.500000000000007105 ) ;
#17535=LINE ( 'NONE', #20970, #4101 ) ;
#17552=ORIENTED_EDGE ( 'NONE', *, *, #19445, .F. ) ;
#17561=SURFACE_STYLE_USAGE ( .BOTH. , #8884 ) ;
#17567=VECTOR ( 'NONE', #11067, 1000.000000000000000 ) ;
#17575=EDGE_CURVE ( 'NONE', #8316, #19257, #1481, .T. ) ;
#17763=ORIENTED_EDGE ( 'NONE', *, *, #11114, .F. ) ;
#17813=FACE_OUTER_BOUND ( 'NONE', #892, .T. ) ;
#17822=DIRECTION ( 'NONE',  ( 1.000000000000000000, -1.387778780781445676E-16, 0.000000000000000000 ) ) ;
#17863=CIRCLE ( 'NONE', #928, 7.500000000000007105 ) ;
#17888=FACE_OUTER_BOUND ( 'NONE', #912, .T. ) ;
#17889=PLANE ( 'NONE',  #8891 ) ;
#17907=ADVANCED_FACE ( 'NONE', ( #21262 ), #1190, .T. ) ;
#17963=DIRECTION ( 'NONE',  ( -1.000000000000000000, 0.000000000000000000, 0.000000000000000000 ) ) ;
#17965=AXIS2_PLACEMENT_3D ( 'NONE', #10047, #1876, #3434 ) ;
#18059=DIRECTION ( 'NONE',  ( 1.000000000000000000, 0.000000000000000000, 0.000000000000000000 ) ) ;
#18088=CYLINDRICAL_SURFACE ( 'NONE', #18518, 7.500000000000007105 ) ;
#18112=DIRECTION ( 'NONE',  ( -1.000000000000000000, 0.000000000000000000, 0.000000000000000000 ) ) ;
#18172=CARTESIAN_POINT ( 'NONE',  ( -27.64582385433943656, -34.13255853780189142, 20.00000000000001776 ) ) ;
#18274=CARTESIAN_POINT ( 'NONE',  ( 148.6725454929228079, -61.68114226949890622, 10.00000000000001599 ) ) ;
#18326=ORIENTED_EDGE ( 'NONE', *, *, #21604, .F. ) ;
#18382=AXIS2_PLACEMENT_3D ( 'NONE', #275, #20664, #13198 ) ;
#18393=EDGE_LOOP ( 'NONE', ( #5656, #17346 ) ) ;
#18462=LINE ( 'NONE', #17119, #6771 ) ;
#18499=DIRECTION ( 'NONE',  ( -0.000000000000000000, -0.000000000000000000, 1.000000000000000000 ) ) ;
#18518=AXIS2_PLACEMENT_3D ( 'NONE', #1456, #14890, #3219 ) ;
#18555=( GEOMETRIC_REPRESENTATION_CONTEXT ( 3 ) GLOBAL_UNCERTAINTY_ASSIGNED_CONTEXT ( ( #20551 ) ) GLOBAL_UNIT_ASSIGNED_CONTEXT ( ( #19886, #2908, #19543 ) ) REPRESENTATION_CONTEXT ( 'NONE', 'WORKASPACE' ) );
#18564=AXIS2_PLACEMENT_3D ( 'NONE', #7833, #16297, #7938 ) ;
#18586=EDGE_LOOP ( 'NONE', ( #18326, #3438, #3202, #5552 ) ) ;
#18612=CARTESIAN_POINT ( 'NONE',  ( -27.64582385433944367, -84.13255853780189852, 5.000000000000018652 ) ) ;
#18685=PLANE ( 'NONE',  #18382 ) ;
#18694=DIRECTION ( 'NONE',  ( 1.387778780781445676E-16, 1.000000000000000000, -0.000000000000000000 ) ) ;
#18726=VECTOR ( 'NONE', #889, 1000.000000000000000 ) ;
#18729=CARTESIAN_POINT ( 'NONE',  ( 11.17254549292281673, -61.68114226949890622, 20.00000000000001776 ) ) ;
#18757=DIRECTION ( 'NONE',  ( -1.000000000000000000, 0.000000000000000000, 0.000000000000000000 ) ) ;
#18771=ORIENTED_EDGE ( 'NONE', *, *, #9116, .F. ) ;
#18813=PLANE ( 'NONE',  #10988 ) ;
#18846=VERTEX_POINT ( 'NONE', #3874 ) ;
#18862=DIRECTION ( 'NONE',  ( -0.000000000000000000, -0.000000000000000000, 1.000000000000000000 ) ) ;
#18876=VECTOR ( 'NONE', #18694, 1000.000000000000000 ) ;
#18877=ORIENTED_EDGE ( 'NONE', *, *, #364, .F. ) ;
#18889=DIRECTION ( 'NONE',  ( 0.000000000000000000, -1.000000000000000000, 0.000000000000000000 ) ) ;
#18987=VECTOR ( 'NONE', #2846, 1000.000000000000000 ) ;
#19066=DIRECTION ( 'NONE',  ( 0.000000000000000000, 0.000000000000000000, 1.000000000000000000 ) ) ;
#19081=VECTOR ( 'NONE', #18862, 1000.000000000000000 ) ;
#19127=DIRECTION ( 'NONE',  ( 1.000000000000000000, 0.000000000000000000, 0.000000000000000000 ) ) ;
#19229=CARTESIAN_POINT ( 'NONE',  ( 148.6725454929228079, -61.68114226949890622, -16.21320343559643717 ) ) ;
#19257=VERTEX_POINT ( 'NONE', #18729 ) ;
#19276=DIRECTION ( 'NONE',  ( -0.000000000000000000, -0.000000000000000000, -1.000000000000000000 ) ) ;
#19281=VECTOR ( 'NONE', #18499, 1000.000000000000000 ) ;
#19360=ORIENTED_EDGE ( 'NONE', *, *, #9116, .T. ) ;
#19372=ADVANCED_FACE ( 'NONE', ( #17813 ), #15840, .F. ) ;
#19424=PLANE ( 'NONE',  #8728 ) ;
#19445=EDGE_CURVE ( 'NONE', #18846, #17048, #1565, .T. ) ;
#19518=ORIENTED_EDGE ( 'NONE', *, *, #16615, .T. ) ;
#19543=( NAMED_UNIT ( * ) SI_UNIT ( $, .STERADIAN. ) SOLID_ANGLE_UNIT ( ) );
#19550=DIRECTION ( 'NONE',  ( -0.000000000000000000, 0.000000000000000000, -1.000000000000000000 ) ) ;
#19597=DIRECTION ( 'NONE',  ( -1.000000000000000000, 0.000000000000000000, 0.000000000000000000 ) ) ;
#19681=EDGE_LOOP ( 'NONE', ( #19978, #9858, #4635, #9095 ) ) ;
#19691=VECTOR ( 'NONE', #9701, 1000.000000000000000 ) ;
#19731=DIRECTION ( 'NONE',  ( 0.000000000000000000, 0.000000000000000000, 1.000000000000000000 ) ) ;
#19734=VERTEX_POINT ( 'NONE', #13192 ) ;
#19760=CARTESIAN_POINT ( 'NONE',  ( 76.17254549292280785, -61.68114226949890622, 10.00000000000001599 ) ) ;
#19768=PLANE ( 'NONE',  #771 ) ;
#19880=FACE_BOUND ( 'NONE', #20634, .T. ) ;
#19886=( LENGTH_UNIT ( ) NAMED_UNIT ( * ) SI_UNIT ( .MILLI., .METRE. ) );
#19892=DIRECTION ( 'NONE',  ( 1.000000000000000000, 0.000000000000000000, 0.000000000000000000 ) ) ;
#19978=ORIENTED_EDGE ( 'NONE', *, *, #21369, .T. ) ;
#20004=EDGE_LOOP ( 'NONE', ( #10613, #12470 ) ) ;
#20210=EDGE_CURVE ( 'NONE', #13608, #12008, #9912, .T. ) ;
#20219=ORIENTED_EDGE ( 'NONE', *, *, #5810, .T. ) ;
#20346=ORIENTED_EDGE ( 'NONE', *, *, #14052, .F. ) ;
#20366=FACE_OUTER_BOUND ( 'NONE', #6959, .T. ) ;
#20463=DIRECTION ( 'NONE',  ( -0.000000000000000000, -0.000000000000000000, 1.000000000000000000 ) ) ;
#20482=AXIS2_PLACEMENT_3D ( 'NONE', #363, #3887, #12252 ) ;
#20526=FACE_OUTER_BOUND ( 'NONE', #6780, .T. ) ;
#20541=EDGE_CURVE ( 'NONE', #5132, #17319, #8485, .T. ) ;
#20551=UNCERTAINTY_MEASURE_WITH_UNIT (LENGTH_MEASURE( 1.000000000000000082E-05 ), #19886, 'distance_accuracy_value', 'NONE');
#20564=DIRECTION ( 'NONE',  ( -1.000000000000000000, 0.000000000000000000, 0.000000000000000000 ) ) ;
#20634=EDGE_LOOP ( 'NONE', ( #11608, #9230 ) ) ;
#20656=CIRCLE ( 'NONE', #6579, 7.500000000000007105 ) ;
#20664=DIRECTION ( 'NONE',  ( -1.000000000000000000, 0.000000000000000000, -0.000000000000000000 ) ) ;
#20688=DIRECTION ( 'NONE',  ( 0.000000000000000000, -1.000000000000000000, -0.000000000000000000 ) ) ;
#20825=LINE ( 'NONE', #10795, #8688 ) ;
#20927=DIRECTION ( 'NONE',  ( -1.000000000000000000, 0.000000000000000000, 0.000000000000000000 ) ) ;
#20970=CARTESIAN_POINT ( 'NONE',  ( 173.3794444120442506, -34.13255853780189142, 20.00000000000001776 ) ) ;
#21024=PRODUCT_DEFINITION_SHAPE ( 'NONE', 'NONE',  #21187 ) ;
#21047=DIRECTION ( 'NONE',  ( -0.000000000000000000, 0.000000000000000000, -1.000000000000000000 ) ) ;
#21066=DIRECTION ( 'NONE',  ( -1.000000000000000000, 0.000000000000000000, 0.000000000000000000 ) ) ;
#21104=LINE ( 'NONE', #4123, #15893 ) ;
#21113=CARTESIAN_POINT ( 'NONE',  ( 5.130598475945862827E-15, 0.000000000000000000, 10.00000000000001599 ) ) ;
#21187=PRODUCT_DEFINITION ( 'UNKNOWN', '', #21476, #15236 ) ;
#21201=ORIENTED_EDGE ( 'NONE', *, *, #17267, .F. ) ;
#21262=FACE_OUTER_BOUND ( 'NONE', #19681, .T. ) ;
#21369=EDGE_CURVE ( 'NONE', #6932, #811, #6494, .T. ) ;
#21377=AXIS2_PLACEMENT_3D ( 'NONE', #6553, #16563, #19892 ) ;
#21381=CARTESIAN_POINT ( 'NONE',  ( 173.3794444120442506, -34.13255853780189142, 5.000000000000018652 ) ) ;
#21476=PRODUCT_DEFINITION_FORMATION_WITH_SPECIFIED_SOURCE ( 'ANY', '', #8013, .NOT_KNOWN. ) ;
#21540=ORIENTED_EDGE ( 'NONE', *, *, #6235, .F. ) ;
#21552=CARTESIAN_POINT ( 'NONE',  ( 91.17254549292282206, -61.68114226949890622, 20.00000000000001776 ) ) ;
#21604=EDGE_CURVE ( 'NONE', #19734, #19257, #16457, .T. ) ;
#21717=COLOUR_RGB ( '', 0.31764706, 0.68627451, 0.89019608) ;
#21735=ORIENTED_EDGE ( 'NONE', *, *, #20541, .T. ) ;
ENDSEC;
END-ISO-10303-21;
